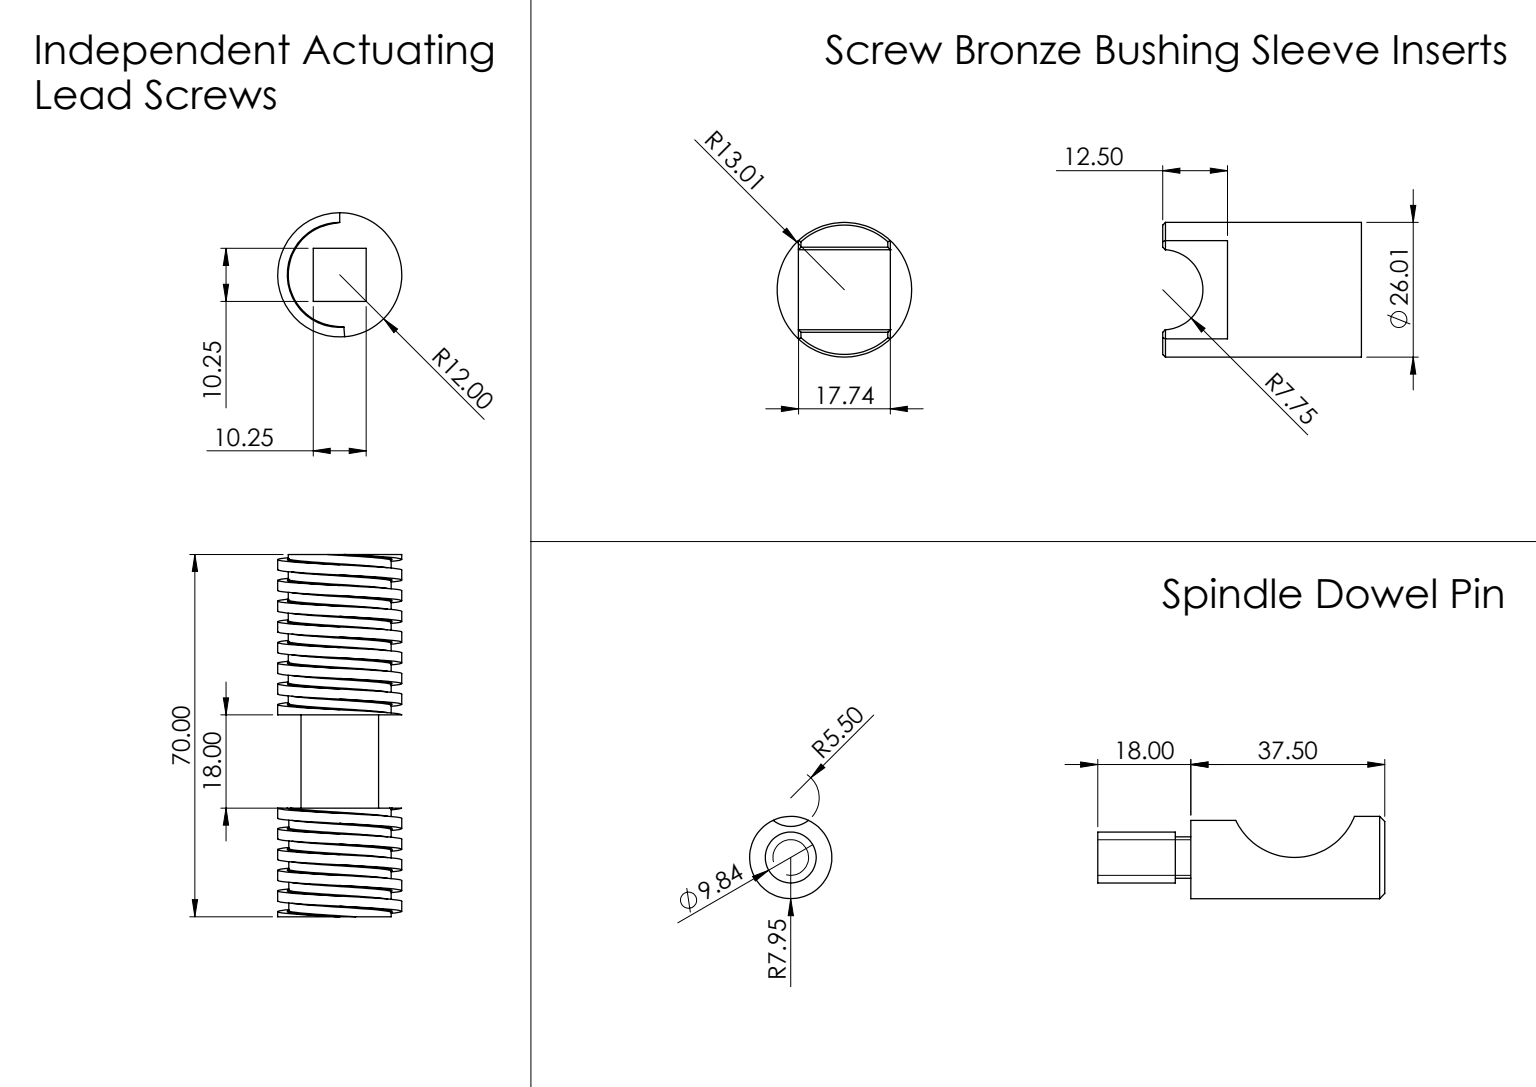
ISO-10303-21;
HEADER;
FILE_DESCRIPTION (('STEP AP214'),
    '1' );
FILE_NAME ('Screw Bronze Bushing Sleeve Inserts.step',
    '2026-10-09T08:48:44',
    ( '' ),
    ( '' ),
    'SwSTEP 2.0',
    'SolidWorks 2026',
    '' );
FILE_SCHEMA (( 'AUTOMOTIVE_DESIGN' ));
ENDSEC;

DATA;
#247=CARTESIAN_POINT ( 'NONE',  ( 0.000000000000000000, 0.000000000000000000, -0.01968503937007903132 ) ) ;
#411=AXIS2_PLACEMENT_3D ( 'NONE', #247, #37306, #45669 ) ;
#485=ORIENTED_EDGE ( 'NONE', *, *, #53883, .T. ) ;
#550=LINE ( 'NONE', #1797, #42889 ) ;
#632=EDGE_CURVE ( 'NONE', #39221, #82812, #83215, .T. ) ;
#636=CARTESIAN_POINT ( 'NONE',  ( -0.3503937007874015630, -0.5120078740157480990, 0.000000000000000000 ) ) ;
#640=ORIENTED_EDGE ( 'NONE', *, *, #71767, .F. ) ;
#1081=ADVANCED_FACE ( 'NONE', ( #25538 ), #52041, .F. ) ;
#1164=( CONVERSION_BASED_UNIT ( 'INCH', #77760 ) LENGTH_UNIT ( ) NAMED_UNIT ( #11550 ) );
#1607=DIRECTION ( 'NONE',  ( 0.000000000000000000, -1.000000000000000000, 0.000000000000000000 ) ) ;
#1797=CARTESIAN_POINT ( 'NONE',  ( -0.5120078740157480990, 6.270288040516270789E-17, -1.512162153811850596 ) ) ;
#1879=VERTEX_POINT ( 'NONE', #17206 ) ;
#1921=ORIENTED_EDGE ( 'NONE', *, *, #43859, .F. ) ;
#2213=CARTESIAN_POINT ( 'NONE',  ( -0.3503937007874015630, 0.3044824468161027586, -0.01968503937007903132 ) ) ;
#2324=CARTESIAN_POINT ( 'NONE',  ( 0.3307086614173228023, 0.3733313776025732333, 0.000000000000000000 ) ) ;
#2406=DIRECTION ( 'NONE',  ( 0.000000000000000000, 0.000000000000000000, 1.000000000000000000 ) ) ;
#2729=EDGE_CURVE ( 'NONE', #71941, #63010, #550, .T. ) ;
#2734=EDGE_CURVE ( 'NONE', #9013, #10037, #67629, .T. ) ;
#2779=ORIENTED_EDGE ( 'NONE', *, *, #31371, .T. ) ;
#2818=EDGE_CURVE ( 'NONE', #52641, #21745, #47224, .T. ) ;
#3260=DIRECTION ( 'NONE',  ( 0.000000000000000000, 0.000000000000000000, -1.000000000000000000 ) ) ;
#3264=DIRECTION ( 'NONE',  ( 1.000000000000000000, 0.000000000000000000, 0.000000000000000000 ) ) ;
#3380=EDGE_CURVE ( 'NONE', #80676, #37563, #44605, .T. ) ;
#3701=CIRCLE ( 'NONE', #66860, 0.3051181102362204856 ) ;
#3736=DIRECTION ( 'NONE',  ( 0.000000000000000000, 0.000000000000000000, -1.000000000000000000 ) ) ;
#3800=CARTESIAN_POINT ( 'NONE',  ( -0.3307086614173228023, -0.3242060844882008741, 0.000000000000000000 ) ) ;
#3854=CARTESIAN_POINT ( 'NONE',  ( -0.3492006680983059108, 0.3045572308828553565, -0.01849200668098333403 ) ) ;
#4023=DIRECTION ( 'NONE',  ( 0.000000000000000000, 0.000000000000000000, 1.000000000000000000 ) ) ;
#4083=CARTESIAN_POINT ( 'NONE',  ( 0.3307086614173228023, -0.3242060844882008741, 0.000000000000000000 ) ) ;
#4228=ORIENTED_EDGE ( 'NONE', *, *, #74315, .F. ) ;
#4282=LINE ( 'NONE', #53548, #31642 ) ;
#4531=VERTEX_POINT ( 'NONE', #67048 ) ;
#4558=DIRECTION ( 'NONE',  ( -1.000000000000000000, 0.000000000000000000, 0.000000000000000000 ) ) ;
#4724=ADVANCED_FACE ( 'NONE', ( #54394 ), #29146, .T. ) ;
#4806=VERTEX_POINT ( 'NONE', #44633 ) ;
#4872=CARTESIAN_POINT ( 'NONE',  ( 0.3499960723095487114, -0.3045081538226084295, -0.01928741089222630808 ) ) ;
#4940=ORIENTED_EDGE ( 'NONE', *, *, #8497, .F. ) ;
#4951=ORIENTED_EDGE ( 'NONE', *, *, #71288, .F. ) ;
#5238=PLANE ( 'NONE',  #54701 ) ;
#5493=FACE_OUTER_BOUND ( 'NONE', #40997, .T. ) ;
#5842=FACE_OUTER_BOUND ( 'NONE', #35715, .T. ) ;
#6102=PLANE ( 'NONE',  #27217 ) ;
#6679=CARTESIAN_POINT ( 'NONE',  ( -0.3499960723095489334, -0.3045081538226084295, -0.01928741089222641911 ) ) ;
#6842=B_SPLINE_CURVE_WITH_KNOTS ( 'NONE', 3,
 ( #38385, #37148, #37971, #63646 ),
 .UNSPECIFIED., .F., .F.,
 ( 4, 4 ),
 ( 0.000000000000000000, 0.0007402370886711635454 ),
 .UNSPECIFIED. ) ;
#7089=VECTOR ( 'NONE', #81498, 39.37007874015748143 ) ;
#7379=EDGE_CURVE ( 'NONE', #70359, #76967, #40027, .T. ) ;
#7622=ORIENTED_EDGE ( 'NONE', *, *, #18824, .T. ) ;
#7793=CARTESIAN_POINT ( 'NONE',  ( 0.000000000000000000, 0.000000000000000000, -0.4921259842519685179 ) ) ;
#7946=DIRECTION ( 'NONE',  ( 0.000000000000000000, -1.000000000000000000, 0.000000000000000000 ) ) ;
#8055=ADVANCED_FACE ( 'NONE', ( #5842 ), #69002, .F. ) ;
#8197=FACE_OUTER_BOUND ( 'NONE', #22520, .T. ) ;
#8497=EDGE_CURVE ( 'NONE', #4531, #11477, #58863, .T. ) ;
#8619=DIRECTION ( 'NONE',  ( -1.000000000000000000, -2.664535259100376091E-15, 0.000000000000000000 ) ) ;
#9013=VERTEX_POINT ( 'NONE', #3854 ) ;
#9053=VECTOR ( 'NONE', #63209, 39.37007874015748143 ) ;
#9136=CARTESIAN_POINT ( 'NONE',  ( 0.000000000000000000, 0.000000000000000000, 0.000000000000000000 ) ) ;
#9233=B_SPLINE_CURVE_WITH_KNOTS ( 'NONE', 3,
 ( #16723, #61316, #15902, #60904 ),
 .UNSPECIFIED., .F., .F.,
 ( 4, 4 ),
 ( 0.000000000000000000, 0.0007402370886711635454 ),
 .UNSPECIFIED. ) ;
#9469=PLANE ( 'NONE',  #56857 ) ;
#9544=LINE ( 'NONE', #80268, #7089 ) ;
#10037=VERTEX_POINT ( 'NONE', #77770 ) ;
#10079=ADVANCED_FACE ( 'NONE', ( #5493 ), #31155, .T. ) ;
#10325=CONICAL_SURFACE ( 'NONE', #21064, 0.4923228346456693938, 0.7853981633974415066 ) ;
#10474=ORIENTED_EDGE ( 'NONE', *, *, #61021, .F. ) ;
#10540=ORIENTED_EDGE ( 'NONE', *, *, #61360, .F. ) ;
#10867=DIRECTION ( 'NONE',  ( 1.000000000000000000, 0.000000000000000000, 0.000000000000000000 ) ) ;
#10874=ORIENTED_EDGE ( 'NONE', *, *, #57015, .F. ) ;
#10877=ORIENTED_EDGE ( 'NONE', *, *, #68192, .T. ) ;
#11012=VECTOR ( 'NONE', #15265, 39.37007874015748143 ) ;
#11153=EDGE_CURVE ( 'NONE', #73823, #76967, #38465, .T. ) ;
#11170=PLANE ( 'NONE',  #81642 ) ;
#11201=CARTESIAN_POINT ( 'NONE',  ( 0.000000000000000000, 0.000000000000000000, -1.512162153811850596 ) ) ;
#11202=( NAMED_UNIT ( * ) PLANE_ANGLE_UNIT ( ) SI_UNIT ( $, .RADIAN. ) );
#11241=DIRECTION ( 'NONE',  ( 0.000000000000000000, 0.000000000000000000, 1.000000000000000000 ) ) ;
#11477=VERTEX_POINT ( 'NONE', #65460 ) ;
#11550=DIMENSIONAL_EXPONENTS ( 1.000000000000000000, 0.000000000000000000, 0.000000000000000000, 0.000000000000000000, 0.000000000000000000, 0.000000000000000000, 0.000000000000000000 ) ;
#11567=FACE_OUTER_BOUND ( 'NONE', #56370, .T. ) ;
#11597=ORIENTED_EDGE ( 'NONE', *, *, #35215, .F. ) ;
#11660=CARTESIAN_POINT ( 'NONE',  ( -0.3503937007874015630, 0.3733313776025731778, -0.01968503937007957602 ) ) ;
#11750=CARTESIAN_POINT ( 'NONE',  ( 0.3438254193631122835, 0.3704879858182167918, -0.01311675794578955577 ) ) ;
#11774=DIRECTION ( 'NONE',  ( -1.000000000000000000, 0.000000000000000000, 0.000000000000000000 ) ) ;
#11815=EDGE_CURVE ( 'NONE', #37563, #63010, #55945, .T. ) ;
#12105=CARTESIAN_POINT ( 'NONE',  ( 0.3503937007874015075, 0.000000000000000000, 0.000000000000000000 ) ) ;
#12271=DIRECTION ( 'NONE',  ( 0.000000000000000000, -1.000000000000000000, 0.000000000000000000 ) ) ;
#12471=CARTESIAN_POINT ( 'NONE',  ( -0.5120078740157480990, 6.270288040516270789E-17, -1.512162153811850596 ) ) ;
#12507=EDGE_LOOP ( 'NONE', ( #80146, #43724, #23079, #52852 ) ) ;
#12856=DIRECTION ( 'NONE',  ( -1.000000000000000000, -0.000000000000000000, -0.000000000000000000 ) ) ;
#12956=CIRCLE ( 'NONE', #21007, 0.5120078740157480990 ) ;
#13033=EDGE_LOOP ( 'NONE', ( #43711, #13139, #1921, #77840, #46885 ) ) ;
#13139=ORIENTED_EDGE ( 'NONE', *, *, #29595, .F. ) ;
#13421=EDGE_CURVE ( 'NONE', #11477, #59797, #78828, .T. ) ;
#13561=EDGE_CURVE ( 'NONE', #4806, #15637, #27878, .T. ) ;
#13564=CARTESIAN_POINT ( 'NONE',  ( 0.000000000000000000, 0.000000000000000000, -1.512162153811850596 ) ) ;
#13846=CARTESIAN_POINT ( 'NONE',  ( -0.3503937007874015630, -0.3044824468161027586, -0.01968503937007903132 ) ) ;
#13895=( BOUNDED_CURVE ( )  B_SPLINE_CURVE ( 3, ( #13846, #6679, #71081, #38665 ),
 .UNSPECIFIED., .F., .F. ) 
 B_SPLINE_CURVE_WITH_KNOTS ( ( 4, 4 ),
 ( 4.647828011067211662, 4.651745756353172112 ),
 .UNSPECIFIED. ) 
 CURVE ( )  GEOMETRIC_REPRESENTATION_ITEM ( )  RATIONAL_B_SPLINE_CURVE ( ( 1.000000000000000000, 0.9999987209397318555, 0.9999987209397318555, 1.000000000000000000 ) ) 
 REPRESENTATION_ITEM ( '' )  );
#14238=CARTESIAN_POINT ( 'NONE',  ( 0.5120078740157480990, 0.000000000000000000, -0.4921259842519685179 ) ) ;
#14350=VECTOR ( 'NONE', #81309, 39.37007874015748143 ) ;
#14364=ORIENTED_EDGE ( 'NONE', *, *, #2818, .T. ) ;
#14443=CARTESIAN_POINT ( 'NONE',  ( 0.3503937007874015630, -0.3733313776025731778, -1.512162153811850596 ) ) ;
#14589=ORIENTED_EDGE ( 'NONE', *, *, #11153, .F. ) ;
#14672=CARTESIAN_POINT ( 'NONE',  ( -0.5120078740157480990, 0.000000000000000000, 0.000000000000000000 ) ) ;
#14915=ORIENTED_EDGE ( 'NONE', *, *, #46568, .T. ) ;
#14932=DIRECTION ( 'NONE',  ( 0.000000000000000000, 0.000000000000000000, -1.000000000000000000 ) ) ;
#15100=PRODUCT_DEFINITION_SHAPE ( 'NONE', 'NONE',  #40864 ) ;
#15227=VECTOR ( 'NONE', #45470, 39.37007874015748143 ) ;
#15265=DIRECTION ( 'NONE',  ( -0.5653208194167064216, 0.6006868920394703437, -0.5653208194167143041 ) ) ;
#15637=VERTEX_POINT ( 'NONE', #58922 ) ;
#15718=ORIENTED_EDGE ( 'NONE', *, *, #78407, .F. ) ;
#15733=VECTOR ( 'NONE', #59443, 39.37007874015748143 ) ;
#15902=CARTESIAN_POINT ( 'NONE',  ( -0.3438254193631122835, -0.3704879858182167918, -0.01311675794578955577 ) ) ;
#16106=CARTESIAN_POINT ( 'NONE',  ( -0.5120078740157480990, 6.270288040516270789E-17, -0.4921259842519685179 ) ) ;
#16394=EDGE_CURVE ( 'NONE', #54726, #60937, #81202, .T. ) ;
#16493=VECTOR ( 'NONE', #24151, 39.37007874015748143 ) ;
#16617=PLANE ( 'NONE',  #80323 ) ;
#16723=CARTESIAN_POINT ( 'NONE',  ( -0.3307086614173228023, -0.3647102339900947787, 0.000000000000000000 ) ) ;
#16777=ORIENTED_EDGE ( 'NONE', *, *, #11153, .T. ) ;
#16967=SURFACE_SIDE_STYLE ('',( #43419 ) ) ;
#17206=CARTESIAN_POINT ( 'NONE',  ( -0.3307086614173228023, 0.3242060844882008741, 0.000000000000000000 ) ) ;
#17217=CARTESIAN_POINT ( 'NONE',  ( -0.3307086614173228023, 0.3051181102362204856, 0.000000000000000000 ) ) ;
#17623=DIRECTION ( 'NONE',  ( 0.000000000000000000, -1.000000000000000000, 0.000000000000000000 ) ) ;
#17962=CONICAL_SURFACE ( 'NONE', #54228, 0.4923228346456693938, 0.7853981633974415066 ) ;
#17971=CARTESIAN_POINT ( 'NONE',  ( -0.3372635250547070807, 0.3676148930005934123, -0.006554863637384360751 ) ) ;
#18121=ADVANCED_FACE ( 'NONE', ( #74689 ), #16617, .T. ) ;
#18322=ORIENTED_EDGE ( 'NONE', *, *, #2729, .F. ) ;
#18325=CARTESIAN_POINT ( 'NONE',  ( -0.3503937007874015630, 0.3733313776025731778, -0.01968503937007957602 ) ) ;
#18730=DIRECTION ( 'NONE',  ( 0.000000000000000000, -1.000000000000000000, 0.000000000000000000 ) ) ;
#18740=DIRECTION ( 'NONE',  ( 0.000000000000000000, 0.000000000000000000, 1.000000000000000000 ) ) ;
#18824=EDGE_CURVE ( 'NONE', #62598, #60937, #32529, .T. ) ;
#19001=LENGTH_MEASURE_WITH_UNIT ( LENGTH_MEASURE( 0.02539999999999999897 ), #20263 );
#19278=EDGE_CURVE ( 'NONE', #65199, #70928, #4282, .T. ) ;
#19544=ORIENTED_EDGE ( 'NONE', *, *, #24864, .F. ) ;
#19666=CARTESIAN_POINT ( 'NONE',  ( -0.3307086614173228023, -0.3647102339900947787, 0.000000000000000000 ) ) ;
#19668=AXIS2_PLACEMENT_3D ( 'NONE', #7793, #66279, #8619 ) ;
#19716=ORIENTED_EDGE ( 'NONE', *, *, #44509, .T. ) ;
#19751=ORIENTED_EDGE ( 'NONE', *, *, #7379, .T. ) ;
#19841=ORIENTED_EDGE ( 'NONE', *, *, #65161, .T. ) ;
#19904=CARTESIAN_POINT ( 'NONE',  ( -0.3492006680983059108, 0.3045572308828553565, -0.01849200668098333403 ) ) ;
#20112=UNCERTAINTY_MEASURE_WITH_UNIT (LENGTH_MEASURE( 1.000000000000000082E-05 ), #1164, 'distance_accuracy_value', 'NONE');
#20263=( LENGTH_UNIT ( ) NAMED_UNIT ( * ) SI_UNIT ( $, .METRE. ) );
#20359=EDGE_CURVE ( 'NONE', #45388, #70359, #33234, .T. ) ;
#20444=VECTOR ( 'NONE', #63989, 39.37007874015748143 ) ;
#20538=CLOSED_SHELL ( 'NONE', ( #66492, #54205, #18121, #44866, #58939, #75378, #40034, #37271, #8055, #1081, #33939, #77308, #21751, #77471, #44868, #41341, #10079, #4724, #73865 ) ) ;
#20699=ORIENTED_EDGE ( 'NONE', *, *, #60494, .F. ) ;
#20979=CARTESIAN_POINT ( 'NONE',  ( 0.3503937007874015630, -0.3733313776025732333, -0.01968503937007903132 ) ) ;
#21007=AXIS2_PLACEMENT_3D ( 'NONE', #26002, #77364, #26428 ) ;
#21064=AXIS2_PLACEMENT_3D ( 'NONE', #80299, #3260, #48273 ) ;
#21164=DIRECTION ( 'NONE',  ( -0.5653208194167064216, -0.6006868920394703437, 0.5653208194167143041 ) ) ;
#21258=EDGE_CURVE ( 'NONE', #10037, #73823, #26237, .T. ) ;
#21745=VERTEX_POINT ( 'NONE', #61700 ) ;
#21751=ADVANCED_FACE ( 'NONE', ( #55368 ), #49057, .T. ) ;
#22098=AXIS2_PLACEMENT_3D ( 'NONE', #9136, #2406, #28064 ) ;
#22520=EDGE_LOOP ( 'NONE', ( #45321, #71370, #51682, #10540, #44365, #19751, #14589 ) ) ;
#22567=ORIENTED_EDGE ( 'NONE', *, *, #71288, .T. ) ;
#22617=( BOUNDED_CURVE ( )  B_SPLINE_CURVE ( 3, ( #46888, #32605, #58268, #65452 ),
 .UNSPECIFIED., .F., .F. ) 
 B_SPLINE_CURVE_WITH_KNOTS ( ( 4, 4 ),
 ( 1.506235357477418768, 1.510153102763379218 ),
 .UNSPECIFIED. ) 
 CURVE ( )  GEOMETRIC_REPRESENTATION_ITEM ( )  RATIONAL_B_SPLINE_CURVE ( ( 1.000000000000000000, 0.9999987209397318555, 0.9999987209397318555, 1.000000000000000000 ) ) 
 REPRESENTATION_ITEM ( '' )  );
#22638=CYLINDRICAL_SURFACE ( 'NONE', #65144, 0.5120078740157480990 ) ;
#22675=DIRECTION ( 'NONE',  ( 1.000000000000000000, -0.000000000000000000, -0.000000000000000000 ) ) ;
#23024=CIRCLE ( 'NONE', #40459, 0.3051181102362204856 ) ;
#23079=ORIENTED_EDGE ( 'NONE', *, *, #76884, .F. ) ;
#23082=LINE ( 'NONE', #68131, #53319 ) ;
#23232=CIRCLE ( 'NONE', #411, 0.5120078740157480990 ) ;
#23298=CARTESIAN_POINT ( 'NONE',  ( -0.3503937007874015630, -0.3733313776025732333, -0.4921259842519685179 ) ) ;
#23334=DIRECTION ( 'NONE',  ( 0.000000000000000000, 0.000000000000000000, 1.000000000000000000 ) ) ;
#23429=EDGE_CURVE ( 'NONE', #80676, #4806, #65323, .T. ) ;
#24151=DIRECTION ( 'NONE',  ( -0.000000000000000000, 1.000000000000000000, -0.000000000000000000 ) ) ;
#24255=B_SPLINE_CURVE_WITH_KNOTS ( 'NONE', 3,
 ( #75633, #17971, #69310, #11660 ),
 .UNSPECIFIED., .F., .F.,
 ( 4, 4 ),
 ( 0.000000000000000000, 0.0007402370886711635454 ),
 .UNSPECIFIED. ) ;
#24262=DIRECTION ( 'NONE',  ( 1.000000000000000000, 0.000000000000000000, 0.000000000000000000 ) ) ;
#24528=EDGE_CURVE ( 'NONE', #43552, #9013, #30649, .T. ) ;
#24605=FACE_OUTER_BOUND ( 'NONE', #45084, .T. ) ;
#24801=CARTESIAN_POINT ( 'NONE',  ( 0.3492006680983059663, 0.3045572308828553565, -0.01849200668098333403 ) ) ;
#24864=EDGE_CURVE ( 'NONE', #82812, #1879, #44488, .T. ) ;
#25044=EDGE_LOOP ( 'NONE', ( #22567, #4228, #49955, #640 ) ) ;
#25114=VERTEX_POINT ( 'NONE', #19666 ) ;
#25406=CARTESIAN_POINT ( 'NONE',  ( -0.5120078740157480990, -0.3045572308828553565, -0.01849200668098333056 ) ) ;
#25458=DIRECTION ( 'NONE',  ( 0.000000000000000000, 0.000000000000000000, -1.000000000000000000 ) ) ;
#25538=FACE_OUTER_BOUND ( 'NONE', #50054, .T. ) ;
#25899=CARTESIAN_POINT ( 'NONE',  ( -0.5120078740157480990, -0.3045572308828553565, -0.01849200668098333403 ) ) ;
#26002=CARTESIAN_POINT ( 'NONE',  ( 0.000000000000000000, 0.000000000000000000, -1.512162153811850596 ) ) ;
#26009=FACE_OUTER_BOUND ( 'NONE', #63041, .T. ) ;
#26173=DIRECTION ( 'NONE',  ( 1.000000000000000000, 0.000000000000000000, 0.000000000000000000 ) ) ;
#26181=DIRECTION ( 'NONE',  ( 1.000000000000000000, 8.881784197001252323E-16, 0.000000000000000000 ) ) ;
#26237=CIRCLE ( 'NONE', #30324, 0.3051181102362204856 ) ;
#26391=ORIENTED_EDGE ( 'NONE', *, *, #44509, .F. ) ;
#26428=DIRECTION ( 'NONE',  ( 1.000000000000000000, 0.000000000000000000, 0.000000000000000000 ) ) ;
#26434=DIRECTION ( 'NONE',  ( -0.7071067811865524577, 0.000000000000000000, 0.7071067811865425767 ) ) ;
#26449=EDGE_LOOP ( 'NONE', ( #64221, #28144, #59396, #59510 ) ) ;
#27138=DIRECTION ( 'NONE',  ( 0.000000000000000000, 1.000000000000000000, 0.000000000000000000 ) ) ;
#27217=AXIS2_PLACEMENT_3D ( 'NONE', #70075, #57437, #62534 ) ;
#27528=ORIENTED_EDGE ( 'NONE', *, *, #2729, .T. ) ;
#27544=PLANE ( 'NONE',  #62696 ) ;
#27815=ORIENTED_EDGE ( 'NONE', *, *, #57015, .T. ) ;
#27878=LINE ( 'NONE', #34194, #14350 ) ;
#27943=ORIENTED_EDGE ( 'NONE', *, *, #49631, .F. ) ;
#28041=ORIENTED_EDGE ( 'NONE', *, *, #19278, .T. ) ;
#28064=DIRECTION ( 'NONE',  ( 1.000000000000000000, 0.000000000000000000, 0.000000000000000000 ) ) ;
#28144=ORIENTED_EDGE ( 'NONE', *, *, #53636, .F. ) ;
#28828=ORIENTED_EDGE ( 'NONE', *, *, #46568, .F. ) ;
#29013=AXIS2_PLACEMENT_3D ( 'NONE', #31248, #45531, #26181 ) ;
#29146=PLANE ( 'NONE',  #51346 ) ;
#29343=DIRECTION ( 'NONE',  ( 0.000000000000000000, 0.000000000000000000, 1.000000000000000000 ) ) ;
#29363=DIRECTION ( 'NONE',  ( 1.000000000000000000, 0.000000000000000000, 0.000000000000000000 ) ) ;
#29450=AXIS2_PLACEMENT_3D ( 'NONE', #63033, #62203, #10867 ) ;
#29595=EDGE_CURVE ( 'NONE', #57099, #39221, #47330, .T. ) ;
#29606=DIRECTION ( 'NONE',  ( 0.000000000000000000, 0.000000000000000000, -1.000000000000000000 ) ) ;
#29807=DIRECTION ( 'NONE',  ( 0.000000000000000000, 0.000000000000000000, 1.000000000000000000 ) ) ;
#30037=VECTOR ( 'NONE', #37862, 39.37007874015748143 ) ;
#30229=( BOUNDED_CURVE ( )  B_SPLINE_CURVE ( 3, ( #37276, #51116, #4872, #62951 ),
 .UNSPECIFIED., .F., .F. ) 
 B_SPLINE_CURVE_WITH_KNOTS ( ( 4, 4 ),
 ( 4.773032204416207236, 4.776949949702167686 ),
 .UNSPECIFIED. ) 
 CURVE ( )  GEOMETRIC_REPRESENTATION_ITEM ( )  RATIONAL_B_SPLINE_CURVE ( ( 1.000000000000000000, 0.9999987209397318555, 0.9999987209397318555, 1.000000000000000000 ) ) 
 REPRESENTATION_ITEM ( '' )  );
#30324=AXIS2_PLACEMENT_3D ( 'NONE', #34793, #34372, #41513 ) ;
#30482=ORIENTED_EDGE ( 'NONE', *, *, #64825, .F. ) ;
#30554=STYLED_ITEM ( 'NONE', ( #36299 ), #61376 ) ;
#30587=CARTESIAN_POINT ( 'NONE',  ( 0.000000000000000000, 0.000000000000000000, 0.000000000000000000 ) ) ;
#30630=DIRECTION ( 'NONE',  ( 1.000000000000000000, 0.000000000000000000, 0.000000000000000000 ) ) ;
#30649=LINE ( 'NONE', #36961, #58621 ) ;
#31077=CARTESIAN_POINT ( 'NONE',  ( 0.3307086614173228023, 0.3647102339900947787, 0.000000000000000000 ) ) ;
#31103=LINE ( 'NONE', #56770, #31526 ) ;
#31155=PLANE ( 'NONE',  #78824 ) ;
#31248=CARTESIAN_POINT ( 'NONE',  ( 0.000000000000000000, 0.000000000000000000, -0.01968503937007903132 ) ) ;
#31371=EDGE_CURVE ( 'NONE', #4531, #38373, #23024, .T. ) ;
#31525=ORIENTED_EDGE ( 'NONE', *, *, #53883, .F. ) ;
#31526=VECTOR ( 'NONE', #58012, 39.37007874015748143 ) ;
#31642=VECTOR ( 'NONE', #48065, 39.37007874015748143 ) ;
#31776=CYLINDRICAL_SURFACE ( 'NONE', #52739, 0.5120078740157480990 ) ;
#31782=ORIENTED_EDGE ( 'NONE', *, *, #78407, .T. ) ;
#31917=COLOUR_RGB ( '', 0.66274510, 0.83137255, 0.94901961) ;
#32529=LINE ( 'NONE', #53127, #51758 ) ;
#32577=APPLICATION_CONTEXT ( 'automotive_design' ) ;
#32605=CARTESIAN_POINT ( 'NONE',  ( 0.3499960723095488224, 0.3045081538226084295, -0.01928741089222631502 ) ) ;
#32614=CARTESIAN_POINT ( 'NONE',  ( -0.3307086614173228023, 0.3647102339900947787, 0.000000000000000000 ) ) ;
#32706=ORIENTED_EDGE ( 'NONE', *, *, #71071, .F. ) ;
#33069=AXIS2_PLACEMENT_3D ( 'NONE', #62960, #12856, #25458 ) ;
#33073=CIRCLE ( 'NONE', #38469, 0.4923228346456693938 ) ;
#33234=LINE ( 'NONE', #39536, #62542 ) ;
#33585=PLANE ( 'NONE',  #42163 ) ;
#33850=CARTESIAN_POINT ( 'NONE',  ( 0.3307086614173228023, 0.3242060844882008741, 0.000000000000000000 ) ) ;
#33939=ADVANCED_FACE ( 'NONE', ( #56917 ), #44280, .F. ) ;
#33964=EDGE_LOOP ( 'NONE', ( #41073, #27528, #54516, #53287, #35377, #82605, #68537, #41174 ) ) ;
#34012=DIRECTION ( 'NONE',  ( 0.000000000000000000, 0.000000000000000000, -1.000000000000000000 ) ) ;
#34031=EDGE_LOOP ( 'NONE', ( #28828, #16777, #485, #61884, #19716, #2779 ) ) ;
#34194=CARTESIAN_POINT ( 'NONE',  ( 0.3503937007874015630, 0.3051181102362204856, -0.01968503937007903132 ) ) ;
#34372=DIRECTION ( 'NONE',  ( -1.000000000000000000, -0.000000000000000000, -0.000000000000000000 ) ) ;
#34683=CARTESIAN_POINT ( 'NONE',  ( 0.3503937007874015630, -0.3733313776025732333, -0.4921259842519685179 ) ) ;
#34707=VECTOR ( 'NONE', #56349, 39.37007874015748143 ) ;
#34793=CARTESIAN_POINT ( 'NONE',  ( -0.3503937007874015630, 0.000000000000000000, 0.000000000000000000 ) ) ;
#35111=CARTESIAN_POINT ( 'NONE',  ( 0.3307086614173228023, -0.3647102339900947787, 0.000000000000000000 ) ) ;
#35215=EDGE_CURVE ( 'NONE', #10037, #80676, #45236, .T. ) ;
#35377=ORIENTED_EDGE ( 'NONE', *, *, #23429, .T. ) ;
#35397=ORIENTED_EDGE ( 'NONE', *, *, #18824, .F. ) ;
#35658=LINE ( 'NONE', #79058, #62284 ) ;
#35715=EDGE_LOOP ( 'NONE', ( #56190, #19841, #67288 ) ) ;
#35717=CYLINDRICAL_SURFACE ( 'NONE', #66809, 0.3051181102362204856 ) ;
#36299=PRESENTATION_STYLE_ASSIGNMENT (( #68307 ) ) ;
#36435=CARTESIAN_POINT ( 'NONE',  ( 0.3307086614173228023, 0.000000000000000000, 0.000000000000000000 ) ) ;
#36860=FACE_OUTER_BOUND ( 'NONE', #26449, .T. ) ;
#36961=CARTESIAN_POINT ( 'NONE',  ( -0.5120078740157480990, 0.3045572308828553565, -0.01849200668098333403 ) ) ;
#37148=CARTESIAN_POINT ( 'NONE',  ( 0.3438254193631122280, -0.3704879858182168473, -0.01311675794578956791 ) ) ;
#37271=ADVANCED_FACE ( 'NONE', ( #8197 ), #27544, .F. ) ;
#37276=CARTESIAN_POINT ( 'NONE',  ( 0.3492006680983059663, -0.3045572308828553565, -0.01849200668098333403 ) ) ;
#37306=DIRECTION ( 'NONE',  ( 0.000000000000000000, 0.000000000000000000, -1.000000000000000000 ) ) ;
#37342=DIMENSIONAL_EXPONENTS ( 1.000000000000000000, 0.000000000000000000, 0.000000000000000000, 0.000000000000000000, 0.000000000000000000, 0.000000000000000000, 0.000000000000000000 ) ;
#37394=CARTESIAN_POINT ( 'NONE',  ( 0.3307086614173228023, -0.3051181102362204856, 0.000000000000000000 ) ) ;
#37563=VERTEX_POINT ( 'NONE', #47307 ) ;
#37809=CARTESIAN_POINT ( 'NONE',  ( 0.3503937007874015630, 0.3733313776025731778, -0.01968503937007957602 ) ) ;
#37820=CARTESIAN_POINT ( 'NONE',  ( -0.6272530615646277896, 0.009110075358399026199, -0.2965444001473090951 ) ) ;
#37862=DIRECTION ( 'NONE',  ( -1.000000000000000000, 0.000000000000000000, 0.000000000000000000 ) ) ;
#37971=CARTESIAN_POINT ( 'NONE',  ( 0.3372635250547070807, -0.3676148930005934123, -0.006554863637384342537 ) ) ;
#38071=ORIENTED_EDGE ( 'NONE', *, *, #71767, .T. ) ;
#38119=LINE ( 'NONE', #25899, #82428 ) ;
#38360=( CONVERSION_BASED_UNIT ( 'INCH', #19001 ) LENGTH_UNIT ( ) NAMED_UNIT ( #37342 ) );
#38373=VERTEX_POINT ( 'NONE', #41072 ) ;
#38385=CARTESIAN_POINT ( 'NONE',  ( 0.3503937007874015630, -0.3733313776025731778, -0.01968503937007957602 ) ) ;
#38465=CIRCLE ( 'NONE', #33069, 0.3051181102362204856 ) ;
#38469=AXIS2_PLACEMENT_3D ( 'NONE', #30587, #11241, #24262 ) ;
#38665=CARTESIAN_POINT ( 'NONE',  ( -0.3492006680983059108, -0.3045572308828553565, -0.01849200668098333403 ) ) ;
#38933=CARTESIAN_POINT ( 'NONE',  ( -0.3503937007874015630, 0.3733313776025732333, -0.01968503937007903132 ) ) ;
#39185=EDGE_LOOP ( 'NONE', ( #27815, #10877, #40575 ) ) ;
#39191=( NAMED_UNIT ( * ) SI_UNIT ( $, .STERADIAN. ) SOLID_ANGLE_UNIT ( ) );
#39221=VERTEX_POINT ( 'NONE', #55754 ) ;
#39536=CARTESIAN_POINT ( 'NONE',  ( -0.3503937007874015630, -0.3733313776025731778, -1.512162153811850596 ) ) ;
#39614=EDGE_LOOP ( 'NONE', ( #31782, #38071, #60148, #48139 ) ) ;
#39657=AXIS2_PLACEMENT_3D ( 'NONE', #70909, #71739, #65008 ) ;
#39903=CARTESIAN_POINT ( 'NONE',  ( 0.000000000000000000, 0.000000000000000000, 0.000000000000000000 ) ) ;
#39995=( GEOMETRIC_REPRESENTATION_CONTEXT ( 3 ) GLOBAL_UNCERTAINTY_ASSIGNED_CONTEXT ( ( #57972 ) ) GLOBAL_UNIT_ASSIGNED_CONTEXT ( ( #38360, #45496, #39191 ) ) REPRESENTATION_CONTEXT ( 'NONE', 'WORKASPACE' ) );
#40027=LINE ( 'NONE', #52212, #44456 ) ;
#40034=ADVANCED_FACE ( 'NONE', ( #66473 ), #35717, .F. ) ;
#40056=EDGE_LOOP ( 'NONE', ( #18322, #64888, #28041, #10874, #51178, #74516, #69344, #57604 ) ) ;
#40252=EDGE_CURVE ( 'NONE', #66145, #4806, #23082, .T. ) ;
#40301=PRODUCT_DEFINITION_CONTEXT ( 'detailed design', #56779, 'design' ) ;
#40310=DIRECTION ( 'NONE',  ( 0.000000000000000000, 0.000000000000000000, 1.000000000000000000 ) ) ;
#40327=CARTESIAN_POINT ( 'NONE',  ( 0.5120078740157480990, 0.000000000000000000, -1.512162153811850596 ) ) ;
#40459=AXIS2_PLACEMENT_3D ( 'NONE', #12105, #30630, #56295 ) ;
#40575=ORIENTED_EDGE ( 'NONE', *, *, #43383, .F. ) ;
#40864=PRODUCT_DEFINITION ( 'UNKNOWN', '', #77247, #40301 ) ;
#40997=EDGE_LOOP ( 'NONE', ( #31525, #77543, #4951, #15718, #14364 ) ) ;
#41072=CARTESIAN_POINT ( 'NONE',  ( 0.3503937007874015075, 0.000000000000000000, -0.3051181102362204856 ) ) ;
#41073=ORIENTED_EDGE ( 'NONE', *, *, #71071, .T. ) ;
#41174=ORIENTED_EDGE ( 'NONE', *, *, #19278, .F. ) ;
#41209=CARTESIAN_POINT ( 'NONE',  ( -0.5120078740157480990, 0.000000000000000000, 0.000000000000000000 ) ) ;
#41341=ADVANCED_FACE ( 'NONE', ( #11567 ), #5238, .F. ) ;
#41513=DIRECTION ( 'NONE',  ( 0.000000000000000000, 8.881784197001252323E-16, -1.000000000000000000 ) ) ;
#41849=DIRECTION ( 'NONE',  ( 0.000000000000000000, 1.000000000000000000, 0.000000000000000000 ) ) ;
#42163=AXIS2_PLACEMENT_3D ( 'NONE', #70628, #26434, #1607 ) ;
#42621=AXIS2_PLACEMENT_3D ( 'NONE', #13564, #59005, #26173 ) ;
#42889=VECTOR ( 'NONE', #59860, 39.37007874015748143 ) ;
#43383=EDGE_CURVE ( 'NONE', #59797, #66145, #55716, .T. ) ;
#43419=SURFACE_STYLE_FILL_AREA ( #55640 ) ;
#43552=VERTEX_POINT ( 'NONE', #24801 ) ;
#43711=ORIENTED_EDGE ( 'NONE', *, *, #76884, .T. ) ;
#43724=ORIENTED_EDGE ( 'NONE', *, *, #632, .F. ) ;
#43783=CARTESIAN_POINT ( 'NONE',  ( -0.3503937007874015630, 0.3733313776025731778, -1.512162153811850596 ) ) ;
#43859=EDGE_CURVE ( 'NONE', #43552, #57099, #9544, .T. ) ;
#44047=ORIENTED_EDGE ( 'NONE', *, *, #74342, .F. ) ;
#44104=CIRCLE ( 'NONE', #77718, 0.5120078740157480990 ) ;
#44280=PLANE ( 'NONE',  #64720 ) ;
#44340=DIRECTION ( 'NONE',  ( -0.000000000000000000, -0.6853444168423467042, -0.7282190812544145908 ) ) ;
#44365=ORIENTED_EDGE ( 'NONE', *, *, #20359, .T. ) ;
#44382=DIRECTION ( 'NONE',  ( 1.000000000000000000, 0.000000000000000000, 0.000000000000000000 ) ) ;
#44456=VECTOR ( 'NONE', #65290, 39.37007874015748143 ) ;
#44488=LINE ( 'NONE', #17217, #68074 ) ;
#44509=EDGE_CURVE ( 'NONE', #62598, #4531, #30229, .T. ) ;
#44605=LINE ( 'NONE', #43783, #20444 ) ;
#44633=CARTESIAN_POINT ( 'NONE',  ( 0.3503937007874015630, 0.3733313776025731778, -0.01968503937007957602 ) ) ;
#44823=DIRECTION ( 'NONE',  ( 1.000000000000000000, -0.000000000000000000, -0.000000000000000000 ) ) ;
#44866=ADVANCED_FACE ( 'NONE', ( #50710 ), #31776, .T. ) ;
#44868=ADVANCED_FACE ( 'NONE', ( #36860 ), #6102, .T. ) ;
#44940=EDGE_CURVE ( 'NONE', #15637, #43552, #22617, .T. ) ;
#45084=EDGE_LOOP ( 'NONE', ( #32706, #20699 ) ) ;
#45236=LINE ( 'NONE', #38933, #46522 ) ;
#45321=ORIENTED_EDGE ( 'NONE', *, *, #21258, .F. ) ;
#45388=VERTEX_POINT ( 'NONE', #23298 ) ;
#45470=DIRECTION ( 'NONE',  ( 1.000000000000000000, -0.000000000000000000, -0.000000000000000000 ) ) ;
#45496=( NAMED_UNIT ( * ) PLANE_ANGLE_UNIT ( ) SI_UNIT ( $, .RADIAN. ) );
#45531=DIRECTION ( 'NONE',  ( 0.000000000000000000, 0.000000000000000000, -1.000000000000000000 ) ) ;
#45669=DIRECTION ( 'NONE',  ( 1.000000000000000000, 0.000000000000000000, 0.000000000000000000 ) ) ;
#46174=DIRECTION ( 'NONE',  ( 0.000000000000000000, -1.000000000000000000, 0.000000000000000000 ) ) ;
#46425=AXIS2_PLACEMENT_3D ( 'NONE', #36435, #57836, #18730 ) ;
#46522=VECTOR ( 'NONE', #27138, 39.37007874015748143 ) ;
#46568=EDGE_CURVE ( 'NONE', #73823, #38373, #71584, .T. ) ;
#46652=PRODUCT ( 'Screw Bronze Bushing Sleeve Inserts', 'Screw Bronze Bushing Sleeve Inserts', '', ( #74669 ) ) ;
#46885=ORIENTED_EDGE ( 'NONE', *, *, #13561, .F. ) ;
#46888=CARTESIAN_POINT ( 'NONE',  ( 0.3503937007874015075, 0.3044824468161027586, -0.01968503937007903132 ) ) ;
#47030=DIRECTION ( 'NONE',  ( 0.000000000000000000, -1.000000000000000000, 0.000000000000000000 ) ) ;
#47224=LINE ( 'NONE', #72913, #11012 ) ;
#47307=CARTESIAN_POINT ( 'NONE',  ( -0.3503937007874015630, 0.3733313776025732333, -0.4921259842519685179 ) ) ;
#47330=LINE ( 'NONE', #2324, #51115 ) ;
#48065=DIRECTION ( 'NONE',  ( 0.000000000000000000, 0.000000000000000000, 1.000000000000000000 ) ) ;
#48101=B_SPLINE_CURVE_WITH_KNOTS ( 'NONE', 3,
 ( #37809, #11750, #62248, #31077 ),
 .UNSPECIFIED., .F., .F.,
 ( 4, 4 ),
 ( 7.561484326770510175E-18, 0.0007402370886711638707 ),
 .UNSPECIFIED. ) ;
#48139=ORIENTED_EDGE ( 'NONE', *, *, #49631, .T. ) ;
#48149=CIRCLE ( 'NONE', #52159, 0.5120078740157480990 ) ;
#48273=DIRECTION ( 'NONE',  ( -1.000000000000000000, 0.000000000000000000, 0.000000000000000000 ) ) ;
#48401=ORIENTED_EDGE ( 'NONE', *, *, #21258, .T. ) ;
#48490=DIRECTION ( 'NONE',  ( 0.7071067811865524577, 0.000000000000000000, 0.7071067811865425767 ) ) ;
#48923=FILL_AREA_STYLE_COLOUR ( '', #31917 ) ;
#48991=DIRECTION ( 'NONE',  ( 1.000000000000000000, 0.000000000000000000, -0.000000000000000000 ) ) ;
#49057=PLANE ( 'NONE',  #46425 ) ;
#49335=LINE ( 'NONE', #69531, #9053 ) ;
#49407=CARTESIAN_POINT ( 'NONE',  ( 0.000000000000000000, 0.000000000000000000, 0.000000000000000000 ) ) ;
#49621=LINE ( 'NONE', #37820, #34707 ) ;
#49631=EDGE_CURVE ( 'NONE', #60937, #52641, #69853, .T. ) ;
#49863=CARTESIAN_POINT ( 'NONE',  ( 0.000000000000000000, 0.000000000000000000, -1.512162153811850596 ) ) ;
#49955=ORIENTED_EDGE ( 'NONE', *, *, #59980, .T. ) ;
#50054=EDGE_LOOP ( 'NONE', ( #79086, #59280, #10474, #56220, #75764, #50575, #52551 ) ) ;
#50062=CARTESIAN_POINT ( 'NONE',  ( 0.3492006680983059663, -0.3045572308828553565, -0.01849200668098333403 ) ) ;
#50575=ORIENTED_EDGE ( 'NONE', *, *, #13421, .T. ) ;
#50710=FACE_OUTER_BOUND ( 'NONE', #40056, .T. ) ;
#50928=AXIS2_PLACEMENT_3D ( 'NONE', #65952, #57937, #77321 ) ;
#51115=VECTOR ( 'NONE', #41849, 39.37007874015748143 ) ;
#51116=CARTESIAN_POINT ( 'NONE',  ( 0.3495983942378627085, -0.3045330818767438275, -0.01888973282054022887 ) ) ;
#51178=ORIENTED_EDGE ( 'NONE', *, *, #13421, .F. ) ;
#51346=AXIS2_PLACEMENT_3D ( 'NONE', #54814, #48490, #12271 ) ;
#51359=CARTESIAN_POINT ( 'NONE',  ( -0.5120078740157480990, 0.000000000000000000, -0.3051181102362204856 ) ) ;
#51394=ORIENTED_EDGE ( 'NONE', *, *, #2818, .F. ) ;
#51666=DIRECTION ( 'NONE',  ( -1.000000000000000000, 0.000000000000000000, 0.000000000000000000 ) ) ;
#51682=ORIENTED_EDGE ( 'NONE', *, *, #3380, .T. ) ;
#51758=VECTOR ( 'NONE', #21164, 39.37007874015748143 ) ;
#52034=MECHANICAL_DESIGN_GEOMETRIC_PRESENTATION_REPRESENTATION('',(#30554),#39995);
#52041=PLANE ( 'NONE',  #50928 ) ;
#52159=AXIS2_PLACEMENT_3D ( 'NONE', #71903, #58422, #52933 ) ;
#52212=CARTESIAN_POINT ( 'NONE',  ( -0.3503937007874015630, -0.3051181102362204856, -0.01968503937007903132 ) ) ;
#52551=ORIENTED_EDGE ( 'NONE', *, *, #43383, .T. ) ;
#52641=VERTEX_POINT ( 'NONE', #3800 ) ;
#52739=AXIS2_PLACEMENT_3D ( 'NONE', #11201, #18740, #44382 ) ;
#52852=ORIENTED_EDGE ( 'NONE', *, *, #23429, .F. ) ;
#52933=DIRECTION ( 'NONE',  ( -1.000000000000000000, 0.000000000000000000, 0.000000000000000000 ) ) ;
#52935=CYLINDRICAL_SURFACE ( 'NONE', #57376, 0.3051181102362204856 ) ;
#53127=CARTESIAN_POINT ( 'NONE',  ( 0.4408028249046178626, -0.2072245076110159345, -0.1100941634872966285 ) ) ;
#53287=ORIENTED_EDGE ( 'NONE', *, *, #3380, .F. ) ;
#53319=VECTOR ( 'NONE', #29807, 39.37007874015748143 ) ;
#53548=CARTESIAN_POINT ( 'NONE',  ( 0.5120078740157480990, 0.000000000000000000, -1.512162153811850596 ) ) ;
#53636=EDGE_CURVE ( 'NONE', #1879, #57099, #31103, .T. ) ;
#53883=EDGE_CURVE ( 'NONE', #76967, #21745, #13895, .T. ) ;
#54205=ADVANCED_FACE ( 'NONE', ( #54613 ), #22638, .T. ) ;
#54228=AXIS2_PLACEMENT_3D ( 'NONE', #39903, #76952, #51666 ) ;
#54394=FACE_OUTER_BOUND ( 'NONE', #72044, .T. ) ;
#54516=ORIENTED_EDGE ( 'NONE', *, *, #11815, .F. ) ;
#54613=FACE_OUTER_BOUND ( 'NONE', #33964, .T. ) ;
#54701=AXIS2_PLACEMENT_3D ( 'NONE', #25406, #44340, #70031 ) ;
#54726=VERTEX_POINT ( 'NONE', #35111 ) ;
#54814=CARTESIAN_POINT ( 'NONE',  ( 0.3307086614173228023, 0.000000000000000000, 0.000000000000000000 ) ) ;
#55267=DIRECTION ( 'NONE',  ( -1.000000000000000000, 0.000000000000000000, -0.000000000000000000 ) ) ;
#55368=FACE_OUTER_BOUND ( 'NONE', #13033, .T. ) ;
#55640=FILL_AREA_STYLE ('',( #48923 ) ) ;
#55716=LINE ( 'NONE', #81426, #16493 ) ;
#55754=CARTESIAN_POINT ( 'NONE',  ( 0.3307086614173228023, 0.3647102339900947787, 0.000000000000000000 ) ) ;
#55945=CIRCLE ( 'NONE', #19668, 0.5120078740157480990 ) ;
#56190=ORIENTED_EDGE ( 'NONE', *, *, #11815, .T. ) ;
#56220=ORIENTED_EDGE ( 'NONE', *, *, #31371, .F. ) ;
#56243=CARTESIAN_POINT ( 'NONE',  ( -0.3503937007874015630, 0.000000000000000000, -0.3051181102362204856 ) ) ;
#56295=DIRECTION ( 'NONE',  ( 0.000000000000000000, 0.000000000000000000, 1.000000000000000000 ) ) ;
#56349=DIRECTION ( 'NONE',  ( -0.5653208194167064216, -0.6006868920394703437, -0.5653208194167143041 ) ) ;
#56370=EDGE_LOOP ( 'NONE', ( #35397, #44047, #51394, #27943 ) ) ;
#56770=CARTESIAN_POINT ( 'NONE',  ( 0.3503937007874016740, 0.3242060844882008741, 0.000000000000000000 ) ) ;
#56779=APPLICATION_CONTEXT ( 'automotive_design' ) ;
#56857=AXIS2_PLACEMENT_3D ( 'NONE', #60805, #23334, #67552 ) ;
#56917=FACE_OUTER_BOUND ( 'NONE', #39185, .T. ) ;
#57015=EDGE_CURVE ( 'NONE', #59797, #70928, #62483, .T. ) ;
#57099=VERTEX_POINT ( 'NONE', #33850 ) ;
#57376=AXIS2_PLACEMENT_3D ( 'NONE', #14672, #58852, #34012 ) ;
#57437=DIRECTION ( 'NONE',  ( 0.000000000000000000, -0.6853444168423467042, 0.7282190812544145908 ) ) ;
#57604=ORIENTED_EDGE ( 'NONE', *, *, #65161, .F. ) ;
#57836=DIRECTION ( 'NONE',  ( 0.7071067811865524577, 0.000000000000000000, 0.7071067811865425767 ) ) ;
#57937=DIRECTION ( 'NONE',  ( -1.000000000000000000, 0.000000000000000000, -0.000000000000000000 ) ) ;
#57972=UNCERTAINTY_MEASURE_WITH_UNIT (LENGTH_MEASURE( 1.000000000000000082E-05 ), #38360, 'distance_accuracy_value', 'NONE');
#58012=DIRECTION ( 'NONE',  ( 1.000000000000000000, 0.000000000000000000, 0.000000000000000000 ) ) ;
#58268=CARTESIAN_POINT ( 'NONE',  ( 0.3495983942378627085, 0.3045330818767438275, -0.01888973282054023581 ) ) ;
#58422=DIRECTION ( 'NONE',  ( 0.000000000000000000, 0.000000000000000000, 1.000000000000000000 ) ) ;
#58621=VECTOR ( 'NONE', #4558, 39.37007874015748143 ) ;
#58806=( LENGTH_UNIT ( ) NAMED_UNIT ( * ) SI_UNIT ( $, .METRE. ) );
#58852=DIRECTION ( 'NONE',  ( 1.000000000000000000, -0.000000000000000000, -0.000000000000000000 ) ) ;
#58863=LINE ( 'NONE', #20979, #60662 ) ;
#58922=CARTESIAN_POINT ( 'NONE',  ( 0.3503937007874015075, 0.3044824468161027586, -0.01968503937007903132 ) ) ;
#58939=ADVANCED_FACE ( 'NONE', ( #24605 ), #11170, .F. ) ;
#59005=DIRECTION ( 'NONE',  ( 0.000000000000000000, 0.000000000000000000, 1.000000000000000000 ) ) ;
#59280=ORIENTED_EDGE ( 'NONE', *, *, #13561, .T. ) ;
#59396=ORIENTED_EDGE ( 'NONE', *, *, #64825, .T. ) ;
#59443=DIRECTION ( 'NONE',  ( -0.000000000000000000, -0.000000000000000000, -1.000000000000000000 ) ) ;
#59510=ORIENTED_EDGE ( 'NONE', *, *, #24528, .F. ) ;
#59797=VERTEX_POINT ( 'NONE', #34683 ) ;
#59860=DIRECTION ( 'NONE',  ( 0.000000000000000000, 0.000000000000000000, 1.000000000000000000 ) ) ;
#59897=DIRECTION ( 'NONE',  ( -1.000000000000000000, 0.000000000000000000, 0.000000000000000000 ) ) ;
#59939=ORIENTED_EDGE ( 'NONE', *, *, #61021, .T. ) ;
#59980=EDGE_CURVE ( 'NONE', #11477, #54726, #6842, .T. ) ;
#60091=CARTESIAN_POINT ( 'NONE',  ( 0.3503937007874015075, 0.000000000000000000, 0.000000000000000000 ) ) ;
#60148=ORIENTED_EDGE ( 'NONE', *, *, #16394, .T. ) ;
#60466=( NAMED_UNIT ( * ) SI_UNIT ( $, .STERADIAN. ) SOLID_ANGLE_UNIT ( ) );
#60494=EDGE_CURVE ( 'NONE', #71941, #65199, #78940, .T. ) ;
#60662=VECTOR ( 'NONE', #7946, 39.37007874015748143 ) ;
#60805=CARTESIAN_POINT ( 'NONE',  ( 0.000000000000000000, 0.000000000000000000, 0.000000000000000000 ) ) ;
#60904=CARTESIAN_POINT ( 'NONE',  ( -0.3503937007874015630, -0.3733313776025731778, -0.01968503937007957602 ) ) ;
#60937=VERTEX_POINT ( 'NONE', #4083 ) ;
#61021=EDGE_CURVE ( 'NONE', #38373, #15637, #3701, .T. ) ;
#61252=ORIENTED_EDGE ( 'NONE', *, *, #24864, .T. ) ;
#61316=CARTESIAN_POINT ( 'NONE',  ( -0.3372635250547070807, -0.3676148930005934123, -0.006554863637384360751 ) ) ;
#61360=EDGE_CURVE ( 'NONE', #45388, #37563, #49335, .T. ) ;
#61376=MANIFOLD_SOLID_BREP ( 'Chamfer1', #20538 ) ;
#61682=DIRECTION ( 'NONE',  ( 1.000000000000000000, 0.000000000000000000, -0.000000000000000000 ) ) ;
#61700=CARTESIAN_POINT ( 'NONE',  ( -0.3492006680983059108, -0.3045572308828553565, -0.01849200668098333403 ) ) ;
#61741=FACE_OUTER_BOUND ( 'NONE', #25044, .T. ) ;
#61884=ORIENTED_EDGE ( 'NONE', *, *, #74342, .T. ) ;
#62203=DIRECTION ( 'NONE',  ( 0.000000000000000000, 0.000000000000000000, 1.000000000000000000 ) ) ;
#62248=CARTESIAN_POINT ( 'NONE',  ( 0.3372635250547070807, 0.3676148930005934123, -0.006554863637384360751 ) ) ;
#62284=VECTOR ( 'NONE', #47030, 39.37007874015748143 ) ;
#62466=FACE_OUTER_BOUND ( 'NONE', #83137, .T. ) ;
#62483=CIRCLE ( 'NONE', #39657, 0.5120078740157480990 ) ;
#62514=ORIENTED_EDGE ( 'NONE', *, *, #44940, .T. ) ;
#62534=DIRECTION ( 'NONE',  ( 1.000000000000000000, -0.000000000000000000, -0.000000000000000000 ) ) ;
#62542=VECTOR ( 'NONE', #64792, 39.37007874015748143 ) ;
#62598=VERTEX_POINT ( 'NONE', #50062 ) ;
#62689=DIRECTION ( 'NONE',  ( -0.000000000000000000, 0.000000000000000000, -1.000000000000000000 ) ) ;
#62696=AXIS2_PLACEMENT_3D ( 'NONE', #636, #72584, #14932 ) ;
#62951=CARTESIAN_POINT ( 'NONE',  ( 0.3503937007874015075, -0.3044824468161027586, -0.01968503937007903132 ) ) ;
#62960=CARTESIAN_POINT ( 'NONE',  ( -0.3503937007874015630, 0.000000000000000000, 0.000000000000000000 ) ) ;
#63010=VERTEX_POINT ( 'NONE', #16106 ) ;
#63033=CARTESIAN_POINT ( 'NONE',  ( 0.000000000000000000, 0.000000000000000000, 0.000000000000000000 ) ) ;
#63041=EDGE_LOOP ( 'NONE', ( #11597, #77215, #30482, #19544, #83191 ) ) ;
#63209=DIRECTION ( 'NONE',  ( -0.000000000000000000, 1.000000000000000000, -0.000000000000000000 ) ) ;
#63646=CARTESIAN_POINT ( 'NONE',  ( 0.3307086614173228023, -0.3647102339900947787, 0.000000000000000000 ) ) ;
#63989=DIRECTION ( 'NONE',  ( -0.000000000000000000, -0.000000000000000000, -1.000000000000000000 ) ) ;
#64221=ORIENTED_EDGE ( 'NONE', *, *, #43859, .T. ) ;
#64720=AXIS2_PLACEMENT_3D ( 'NONE', #69970, #29606, #55267 ) ;
#64792=DIRECTION ( 'NONE',  ( 0.000000000000000000, 0.000000000000000000, 1.000000000000000000 ) ) ;
#64825=EDGE_CURVE ( 'NONE', #1879, #9013, #49621, .T. ) ;
#64888=ORIENTED_EDGE ( 'NONE', *, *, #60494, .T. ) ;
#65008=DIRECTION ( 'NONE',  ( -1.000000000000000000, 0.000000000000000000, 0.000000000000000000 ) ) ;
#65120=( GEOMETRIC_REPRESENTATION_CONTEXT ( 3 ) GLOBAL_UNCERTAINTY_ASSIGNED_CONTEXT ( ( #20112 ) ) GLOBAL_UNIT_ASSIGNED_CONTEXT ( ( #1164, #11202, #60466 ) ) REPRESENTATION_CONTEXT ( 'NONE', 'WORKASPACE' ) );
#65144=AXIS2_PLACEMENT_3D ( 'NONE', #79908, #66857, #29363 ) ;
#65161=EDGE_CURVE ( 'NONE', #63010, #45388, #48149, .T. ) ;
#65199=VERTEX_POINT ( 'NONE', #40327 ) ;
#65290=DIRECTION ( 'NONE',  ( 0.000000000000000000, 1.000000000000000000, 0.000000000000000000 ) ) ;
#65323=CIRCLE ( 'NONE', #29013, 0.5120078740157480990 ) ;
#65452=CARTESIAN_POINT ( 'NONE',  ( 0.3492006680983059663, 0.3045572308828553565, -0.01849200668098333403 ) ) ;
#65460=CARTESIAN_POINT ( 'NONE',  ( 0.3503937007874015630, -0.3733313776025731778, -0.01968503937007957602 ) ) ;
#65952=CARTESIAN_POINT ( 'NONE',  ( 0.3503937007874015630, -0.5120078740157480990, 0.000000000000000000 ) ) ;
#65973=DIRECTION ( 'NONE',  ( -0.7071067811865524577, 0.000000000000000000, 0.7071067811865425767 ) ) ;
#66012=AXIS2_PLACEMENT_3D ( 'NONE', #76973, #62689, #11774 ) ;
#66145=VERTEX_POINT ( 'NONE', #69319 ) ;
#66279=DIRECTION ( 'NONE',  ( 0.000000000000000000, 0.000000000000000000, 1.000000000000000000 ) ) ;
#66473=FACE_OUTER_BOUND ( 'NONE', #34031, .T. ) ;
#66492=ADVANCED_FACE ( 'NONE', ( #72325 ), #52935, .F. ) ;
#66809=AXIS2_PLACEMENT_3D ( 'NONE', #41209, #22675, #3736 ) ;
#66857=DIRECTION ( 'NONE',  ( 0.000000000000000000, 0.000000000000000000, 1.000000000000000000 ) ) ;
#66860=AXIS2_PLACEMENT_3D ( 'NONE', #60091, #3264, #29343 ) ;
#67048=CARTESIAN_POINT ( 'NONE',  ( 0.3503937007874015075, -0.3044824468161027586, -0.01968503937007903132 ) ) ;
#67288=ORIENTED_EDGE ( 'NONE', *, *, #61360, .T. ) ;
#67552=DIRECTION ( 'NONE',  ( 1.000000000000000000, 0.000000000000000000, -0.000000000000000000 ) ) ;
#67629=( BOUNDED_CURVE ( )  B_SPLINE_CURVE ( 3, ( #19904, #71667, #72502, #2213 ),
 .UNSPECIFIED., .F., .F. ) 
 B_SPLINE_CURVE_WITH_KNOTS ( ( 4, 4 ),
 ( 1.631439550826413676, 1.635357296112374570 ),
 .UNSPECIFIED. ) 
 CURVE ( )  GEOMETRIC_REPRESENTATION_ITEM ( )  RATIONAL_B_SPLINE_CURVE ( ( 1.000000000000000000, 0.9999987209397318555, 0.9999987209397318555, 1.000000000000000000 ) ) 
 REPRESENTATION_ITEM ( '' )  );
#67933=SHAPE_DEFINITION_REPRESENTATION ( #15100, #82043 ) ;
#68074=VECTOR ( 'NONE', #17623, 39.37007874015748143 ) ;
#68131=CARTESIAN_POINT ( 'NONE',  ( 0.3503937007874015630, 0.3733313776025731778, -1.512162153811850596 ) ) ;
#68192=EDGE_CURVE ( 'NONE', #70928, #66145, #44104, .T. ) ;
#68307=SURFACE_STYLE_USAGE ( .BOTH. , #16967 ) ;
#68537=ORIENTED_EDGE ( 'NONE', *, *, #68192, .F. ) ;
#68561=ADVANCED_BREP_SHAPE_REPRESENTATION ( '', ( #61376, #22098 ), #65120 ) ;
#69002=PLANE ( 'NONE',  #66012 ) ;
#69310=CARTESIAN_POINT ( 'NONE',  ( -0.3438254193631122835, 0.3704879858182167918, -0.01311675794578955577 ) ) ;
#69319=CARTESIAN_POINT ( 'NONE',  ( 0.3503937007874015630, 0.3733313776025732333, -0.4921259842519685179 ) ) ;
#69344=ORIENTED_EDGE ( 'NONE', *, *, #20359, .F. ) ;
#69531=CARTESIAN_POINT ( 'NONE',  ( -0.3503937007874015630, -0.5120078740157480990, -0.4921259842519685179 ) ) ;
#69853=LINE ( 'NONE', #70683, #30037 ) ;
#69970=CARTESIAN_POINT ( 'NONE',  ( 0.3503937007874015630, -0.5120078740157480990, -0.4921259842519685179 ) ) ;
#70031=DIRECTION ( 'NONE',  ( 1.000000000000000000, -0.000000000000000000, -0.000000000000000000 ) ) ;
#70075=CARTESIAN_POINT ( 'NONE',  ( -0.5120078740157480990, 0.3045572308828553565, -0.01849200668098333056 ) ) ;
#70356=ORIENTED_EDGE ( 'NONE', *, *, #59980, .F. ) ;
#70359=VERTEX_POINT ( 'NONE', #76946 ) ;
#70496=ORIENTED_EDGE ( 'NONE', *, *, #24528, .T. ) ;
#70628=CARTESIAN_POINT ( 'NONE',  ( -0.3503937007874015630, -0.5120078740157480990, -0.01968503937007903132 ) ) ;
#70683=CARTESIAN_POINT ( 'NONE',  ( -0.3503937007874015630, -0.3242060844882008741, 0.000000000000000000 ) ) ;
#70864=VECTOR ( 'NONE', #82027, 39.37007874015748143 ) ;
#70909=CARTESIAN_POINT ( 'NONE',  ( 0.000000000000000000, 0.000000000000000000, -0.4921259842519685179 ) ) ;
#70928=VERTEX_POINT ( 'NONE', #14238 ) ;
#71071=EDGE_CURVE ( 'NONE', #65199, #71941, #12956, .T. ) ;
#71081=CARTESIAN_POINT ( 'NONE',  ( -0.3495983942378629306, -0.3045330818767438275, -0.01888973282054034336 ) ) ;
#71288=EDGE_CURVE ( 'NONE', #25114, #70359, #9233, .T. ) ;
#71370=ORIENTED_EDGE ( 'NONE', *, *, #35215, .T. ) ;
#71448=CARTESIAN_POINT ( 'NONE',  ( -0.3503937007874015630, -0.5120078740157480990, -0.01968503937007903132 ) ) ;
#71584=LINE ( 'NONE', #51359, #15227 ) ;
#71604=ORIENTED_EDGE ( 'NONE', *, *, #632, .T. ) ;
#71667=CARTESIAN_POINT ( 'NONE',  ( -0.3495983942378627640, 0.3045330818767438275, -0.01888973282054017683 ) ) ;
#71739=DIRECTION ( 'NONE',  ( -0.000000000000000000, -0.000000000000000000, 1.000000000000000000 ) ) ;
#71767=EDGE_CURVE ( 'NONE', #25114, #54726, #33073, .T. ) ;
#71791=EDGE_CURVE ( 'NONE', #82812, #80676, #24255, .T. ) ;
#71903=CARTESIAN_POINT ( 'NONE',  ( 0.000000000000000000, 0.000000000000000000, -0.4921259842519685179 ) ) ;
#71941=VERTEX_POINT ( 'NONE', #12471 ) ;
#72044=EDGE_LOOP ( 'NONE', ( #7622, #81985, #70356, #4940, #26391 ) ) ;
#72325=FACE_OUTER_BOUND ( 'NONE', #77330, .T. ) ;
#72502=CARTESIAN_POINT ( 'NONE',  ( -0.3499960723095488779, 0.3045081538226084295, -0.01928741089222630462 ) ) ;
#72584=DIRECTION ( 'NONE',  ( 1.000000000000000000, 0.000000000000000000, 0.000000000000000000 ) ) ;
#72913=CARTESIAN_POINT ( 'NONE',  ( -0.4012318369997560086, -0.2492710286714439338, -0.07052317558243419160 ) ) ;
#72951=CARTESIAN_POINT ( 'NONE',  ( 0.000000000000000000, 0.000000000000000000, -0.4921259842519685179 ) ) ;
#73529=SHAPE_REPRESENTATION_RELATIONSHIP ( 'NONE' , 'NONE' ,  #82043, #68561 ) ;
#73823=VERTEX_POINT ( 'NONE', #56243 ) ;
#73865=ADVANCED_FACE ( 'NONE', ( #61741 ), #10325, .T. ) ;
#74315=EDGE_CURVE ( 'NONE', #11477, #70359, #23232, .T. ) ;
#74342=EDGE_CURVE ( 'NONE', #21745, #62598, #38119, .T. ) ;
#74516=ORIENTED_EDGE ( 'NONE', *, *, #74315, .T. ) ;
#74669=PRODUCT_CONTEXT ( 'NONE', #32577, 'mechanical' ) ;
#74689=FACE_OUTER_BOUND ( 'NONE', #39614, .T. ) ;
#75378=ADVANCED_FACE ( 'NONE', ( #62466 ), #9469, .T. ) ;
#75633=CARTESIAN_POINT ( 'NONE',  ( -0.3307086614173228023, 0.3647102339900947787, 0.000000000000000000 ) ) ;
#75764=ORIENTED_EDGE ( 'NONE', *, *, #8497, .T. ) ;
#76884=EDGE_CURVE ( 'NONE', #4806, #39221, #48101, .T. ) ;
#76946=CARTESIAN_POINT ( 'NONE',  ( -0.3503937007874015630, -0.3733313776025731778, -0.01968503937007957602 ) ) ;
#76952=DIRECTION ( 'NONE',  ( 0.000000000000000000, 0.000000000000000000, -1.000000000000000000 ) ) ;
#76967=VERTEX_POINT ( 'NONE', #82852 ) ;
#76973=CARTESIAN_POINT ( 'NONE',  ( -0.3503937007874015630, -0.5120078740157480990, -0.4921259842519685179 ) ) ;
#77215=ORIENTED_EDGE ( 'NONE', *, *, #2734, .F. ) ;
#77247=PRODUCT_DEFINITION_FORMATION_WITH_SPECIFIED_SOURCE ( 'ANY', '', #46652, .NOT_KNOWN. ) ;
#77308=ADVANCED_FACE ( 'NONE', ( #77794 ), #17962, .T. ) ;
#77321=DIRECTION ( 'NONE',  ( -0.000000000000000000, 0.000000000000000000, 1.000000000000000000 ) ) ;
#77330=EDGE_LOOP ( 'NONE', ( #48401, #14915, #59939, #62514, #70496, #79390 ) ) ;
#77364=DIRECTION ( 'NONE',  ( 0.000000000000000000, 0.000000000000000000, 1.000000000000000000 ) ) ;
#77471=ADVANCED_FACE ( 'NONE', ( #26009 ), #33585, .T. ) ;
#77543=ORIENTED_EDGE ( 'NONE', *, *, #7379, .F. ) ;
#77718=AXIS2_PLACEMENT_3D ( 'NONE', #72951, #78865, #59897 ) ;
#77760=LENGTH_MEASURE_WITH_UNIT ( LENGTH_MEASURE( 0.02539999999999999897 ), #58806 );
#77770=CARTESIAN_POINT ( 'NONE',  ( -0.3503937007874015630, 0.3044824468161027586, -0.01968503937007903132 ) ) ;
#77794=FACE_OUTER_BOUND ( 'NONE', #12507, .T. ) ;
#77840=ORIENTED_EDGE ( 'NONE', *, *, #44940, .F. ) ;
#78407=EDGE_CURVE ( 'NONE', #52641, #25114, #35658, .T. ) ;
#78824=AXIS2_PLACEMENT_3D ( 'NONE', #71448, #65973, #46174 ) ;
#78828=LINE ( 'NONE', #14443, #15733 ) ;
#78865=DIRECTION ( 'NONE',  ( -0.000000000000000000, -0.000000000000000000, 1.000000000000000000 ) ) ;
#78940=CIRCLE ( 'NONE', #42621, 0.5120078740157480990 ) ;
#79058=CARTESIAN_POINT ( 'NONE',  ( -0.3307086614173228023, -0.3733313776025732333, 0.000000000000000000 ) ) ;
#79086=ORIENTED_EDGE ( 'NONE', *, *, #40252, .T. ) ;
#79390=ORIENTED_EDGE ( 'NONE', *, *, #2734, .T. ) ;
#79908=CARTESIAN_POINT ( 'NONE',  ( 0.000000000000000000, 0.000000000000000000, -1.512162153811850596 ) ) ;
#80146=ORIENTED_EDGE ( 'NONE', *, *, #71791, .F. ) ;
#80268=CARTESIAN_POINT ( 'NONE',  ( 0.4408028249046178626, 0.2072245076110159345, -0.1100941634872966285 ) ) ;
#80299=CARTESIAN_POINT ( 'NONE',  ( 0.000000000000000000, 0.000000000000000000, 0.000000000000000000 ) ) ;
#80323=AXIS2_PLACEMENT_3D ( 'NONE', #49407, #40310, #48991 ) ;
#80676=VERTEX_POINT ( 'NONE', #18325 ) ;
#81161=ORIENTED_EDGE ( 'NONE', *, *, #53636, .T. ) ;
#81202=LINE ( 'NONE', #37394, #70864 ) ;
#81309=DIRECTION ( 'NONE',  ( 0.000000000000000000, -1.000000000000000000, 0.000000000000000000 ) ) ;
#81426=CARTESIAN_POINT ( 'NONE',  ( 0.3503937007874015630, -0.5120078740157480990, -0.4921259842519685179 ) ) ;
#81498=DIRECTION ( 'NONE',  ( -0.5653208194167064216, 0.6006868920394703437, 0.5653208194167143041 ) ) ;
#81642=AXIS2_PLACEMENT_3D ( 'NONE', #49863, #4023, #61682 ) ;
#81985=ORIENTED_EDGE ( 'NONE', *, *, #16394, .F. ) ;
#82004=ORIENTED_EDGE ( 'NONE', *, *, #29595, .T. ) ;
#82027=DIRECTION ( 'NONE',  ( 0.000000000000000000, 1.000000000000000000, 0.000000000000000000 ) ) ;
#82043=SHAPE_REPRESENTATION ( 'Screw Bronze Bushing Sleeve Inserts', ( #22098 ), #65120 ) ;
#82428=VECTOR ( 'NONE', #44823, 39.37007874015748143 ) ;
#82605=ORIENTED_EDGE ( 'NONE', *, *, #40252, .F. ) ;
#82812=VERTEX_POINT ( 'NONE', #32614 ) ;
#82852=CARTESIAN_POINT ( 'NONE',  ( -0.3503937007874015630, -0.3044824468161027586, -0.01968503937007903132 ) ) ;
#83137=EDGE_LOOP ( 'NONE', ( #61252, #81161, #82004, #71604 ) ) ;
#83191=ORIENTED_EDGE ( 'NONE', *, *, #71791, .T. ) ;
#83215=CIRCLE ( 'NONE', #29450, 0.4923228346456693938 ) ;
ENDSEC;
END-ISO-10303-21;
